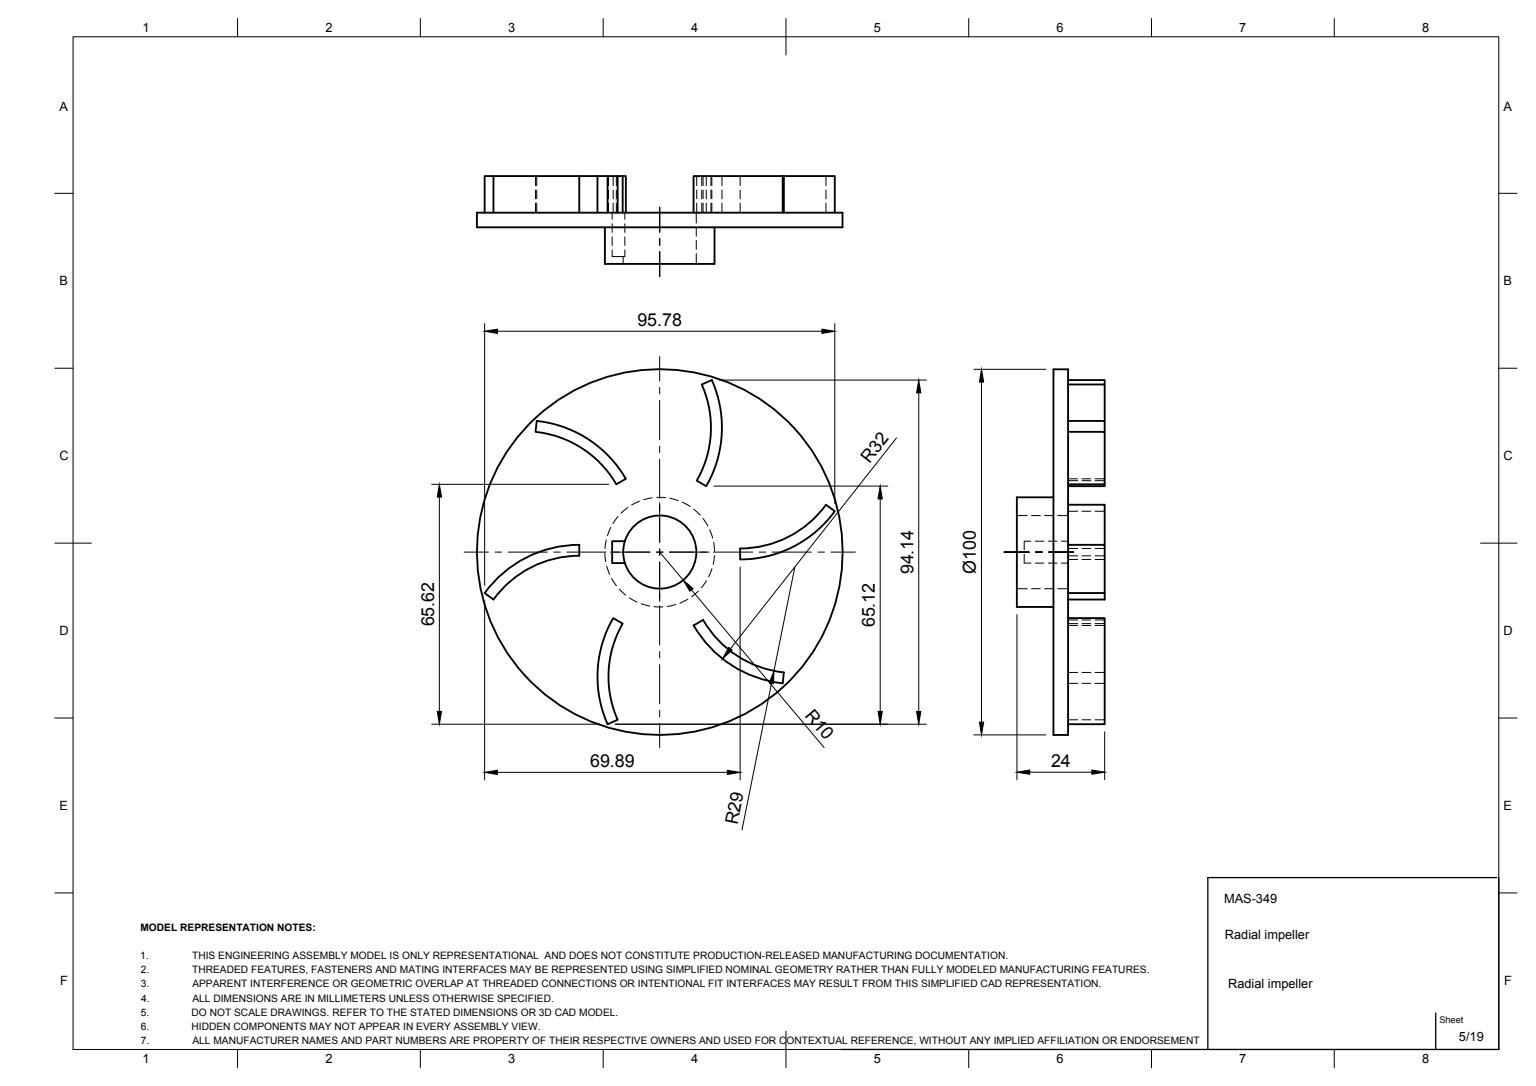
ISO-10303-21;
HEADER;
/* Generated by software containing ST-Developer
 * from STEP Tools, Inc. (www.steptools.com) 
 */

FILE_DESCRIPTION(
/* description */ ('Independent two-stage semi-open centrifugal-pump CAD. Shared impeller
s, open-machinable return casings, removable diaphragms, bronze wear/j
ournal rings, volume-preserving seal instances, retained keyed shaft, 
opposed mechanical face rings and partly threaded tie hardware. Native
 shaft rotation. Geometric topology/clearance only; flow/head/efficien
cy, pressure, cavitation, balance, preload, face loading and secondary
 seal fits/bonds, material/thermal/tolerance selection and life unassi
gned. External drive, coupling, anchors and piping bolts omitted.'),
/* implementation_level */ '2;1');

FILE_NAME(
/* name */ 'Radial impeller.step',
/* time_stamp */ '2026-11-08T18:06:32-08:00',
/* author */ (''),
/* organization */ (''),
/* preprocessor_version */ 'ST-DEVELOPER v20.2',
/* originating_system */ 'Autodesk Translation Framework v15.17.0.0',
/* authorisation */ '');

FILE_SCHEMA (('AUTOMOTIVE_DESIGN { 1 0 10303 214 3 1 1 }'));
ENDSEC;

DATA;
#10=MECHANICAL_DESIGN_GEOMETRIC_PRESENTATION_REPRESENTATION('',(#395),#16687);
#357=SHAPE_REPRESENTATION_RELATIONSHIP('SRR','None',#16766,#376);
#376=ADVANCED_BREP_SHAPE_REPRESENTATION('',(#414),#16670);
#395=STYLED_ITEM('',(#16870),#414);
#414=MANIFOLD_SOLID_BREP('Body1',#6114);
#466=FACE_BOUND('',#1139,.T.);
#467=FACE_BOUND('',#1140,.T.);
#468=FACE_BOUND('',#1141,.T.);
#469=FACE_BOUND('',#1142,.T.);
#470=FACE_BOUND('',#1143,.T.);
#471=FACE_BOUND('',#1144,.T.);
#472=FACE_BOUND('',#1145,.T.);
#473=FACE_BOUND('',#1178,.T.);
#474=FACE_BOUND('',#1182,.T.);
#587=PLANE('',#6481);
#588=PLANE('',#6482);
#589=PLANE('',#6483);
#590=PLANE('',#6484);
#591=PLANE('',#6486);
#592=PLANE('',#6504);
#593=PLANE('',#6507);
#594=PLANE('',#6508);
#595=PLANE('',#6511);
#596=PLANE('',#6514);
#597=PLANE('',#6515);
#598=PLANE('',#6518);
#599=PLANE('',#6521);
#600=PLANE('',#6522);
#601=PLANE('',#6525);
#602=PLANE('',#6528);
#603=PLANE('',#6529);
#604=PLANE('',#6532);
#605=PLANE('',#6535);
#606=PLANE('',#6536);
#607=PLANE('',#6539);
#608=PLANE('',#6542);
#609=PLANE('',#6543);
#610=PLANE('',#6547);
#611=PLANE('',#6552);
#752=FACE_OUTER_BOUND('',#1134,.T.);
#753=FACE_OUTER_BOUND('',#1135,.T.);
#754=FACE_OUTER_BOUND('',#1136,.T.);
#755=FACE_OUTER_BOUND('',#1137,.T.);
#756=FACE_OUTER_BOUND('',#1138,.T.);
#757=FACE_OUTER_BOUND('',#1146,.T.);
#758=FACE_OUTER_BOUND('',#1147,.T.);
#759=FACE_OUTER_BOUND('',#1148,.T.);
#760=FACE_OUTER_BOUND('',#1149,.T.);
#761=FACE_OUTER_BOUND('',#1150,.T.);
#762=FACE_OUTER_BOUND('',#1151,.T.);
#763=FACE_OUTER_BOUND('',#1152,.T.);
#764=FACE_OUTER_BOUND('',#1153,.T.);
#765=FACE_OUTER_BOUND('',#1154,.T.);
#766=FACE_OUTER_BOUND('',#1155,.T.);
#767=FACE_OUTER_BOUND('',#1156,.T.);
#768=FACE_OUTER_BOUND('',#1157,.T.);
#769=FACE_OUTER_BOUND('',#1158,.T.);
#770=FACE_OUTER_BOUND('',#1159,.T.);
#771=FACE_OUTER_BOUND('',#1160,.T.);
#772=FACE_OUTER_BOUND('',#1161,.T.);
#773=FACE_OUTER_BOUND('',#1162,.T.);
#774=FACE_OUTER_BOUND('',#1163,.T.);
#775=FACE_OUTER_BOUND('',#1164,.T.);
#776=FACE_OUTER_BOUND('',#1165,.T.);
#777=FACE_OUTER_BOUND('',#1166,.T.);
#778=FACE_OUTER_BOUND('',#1167,.T.);
#779=FACE_OUTER_BOUND('',#1168,.T.);
#780=FACE_OUTER_BOUND('',#1169,.T.);
#781=FACE_OUTER_BOUND('',#1170,.T.);
#782=FACE_OUTER_BOUND('',#1171,.T.);
#783=FACE_OUTER_BOUND('',#1172,.T.);
#784=FACE_OUTER_BOUND('',#1173,.T.);
#785=FACE_OUTER_BOUND('',#1174,.T.);
#786=FACE_OUTER_BOUND('',#1175,.T.);
#787=FACE_OUTER_BOUND('',#1176,.T.);
#788=FACE_OUTER_BOUND('',#1177,.T.);
#789=FACE_OUTER_BOUND('',#1179,.T.);
#790=FACE_OUTER_BOUND('',#1180,.T.);
#791=FACE_OUTER_BOUND('',#1181,.T.);
#1134=EDGE_LOOP('',(#4209,#4210,#4211,#4212));
#1135=EDGE_LOOP('',(#4213,#4214,#4215,#4216));
#1136=EDGE_LOOP('',(#4217,#4218,#4219,#4220));
#1137=EDGE_LOOP('',(#4221,#4222,#4223,#4224));
#1138=EDGE_LOOP('',(#4225));
#1139=EDGE_LOOP('',(#4226,#4227,#4228,#4229));
#1140=EDGE_LOOP('',(#4230,#4231,#4232,#4233));
#1141=EDGE_LOOP('',(#4234,#4235,#4236,#4237));
#1142=EDGE_LOOP('',(#4238,#4239,#4240,#4241));
#1143=EDGE_LOOP('',(#4242,#4243,#4244,#4245));
#1144=EDGE_LOOP('',(#4246,#4247,#4248,#4249));
#1145=EDGE_LOOP('',(#4250,#4251,#4252,#4253,#4254));
#1146=EDGE_LOOP('',(#4255,#4256,#4257,#4258));
#1147=EDGE_LOOP('',(#4259,#4260,#4261,#4262));
#1148=EDGE_LOOP('',(#4263,#4264,#4265,#4266));
#1149=EDGE_LOOP('',(#4267,#4268,#4269,#4270));
#1150=EDGE_LOOP('',(#4271,#4272,#4273,#4274));
#1151=EDGE_LOOP('',(#4275,#4276,#4277,#4278));
#1152=EDGE_LOOP('',(#4279,#4280,#4281,#4282));
#1153=EDGE_LOOP('',(#4283,#4284,#4285,#4286));
#1154=EDGE_LOOP('',(#4287,#4288,#4289,#4290));
#1155=EDGE_LOOP('',(#4291,#4292,#4293,#4294));
#1156=EDGE_LOOP('',(#4295,#4296,#4297,#4298));
#1157=EDGE_LOOP('',(#4299,#4300,#4301,#4302));
#1158=EDGE_LOOP('',(#4303,#4304,#4305,#4306));
#1159=EDGE_LOOP('',(#4307,#4308,#4309,#4310));
#1160=EDGE_LOOP('',(#4311,#4312,#4313,#4314));
#1161=EDGE_LOOP('',(#4315,#4316,#4317,#4318));
#1162=EDGE_LOOP('',(#4319,#4320,#4321,#4322));
#1163=EDGE_LOOP('',(#4323,#4324,#4325,#4326));
#1164=EDGE_LOOP('',(#4327,#4328,#4329,#4330));
#1165=EDGE_LOOP('',(#4331,#4332,#4333,#4334));
#1166=EDGE_LOOP('',(#4335,#4336,#4337,#4338));
#1167=EDGE_LOOP('',(#4339,#4340,#4341,#4342));
#1168=EDGE_LOOP('',(#4343,#4344,#4345,#4346));
#1169=EDGE_LOOP('',(#4347,#4348,#4349,#4350));
#1170=EDGE_LOOP('',(#4351,#4352,#4353,#4354));
#1171=EDGE_LOOP('',(#4355,#4356,#4357,#4358));
#1172=EDGE_LOOP('',(#4359,#4360,#4361,#4362));
#1173=EDGE_LOOP('',(#4363,#4364,#4365,#4366));
#1174=EDGE_LOOP('',(#4367,#4368,#4369,#4370));
#1175=EDGE_LOOP('',(#4371,#4372,#4373,#4374));
#1176=EDGE_LOOP('',(#4375,#4376,#4377,#4378));
#1177=EDGE_LOOP('',(#4379));
#1178=EDGE_LOOP('',(#4380));
#1179=EDGE_LOOP('',(#4381,#4382,#4383,#4384,#4385,#4386,#4387,#4388));
#1180=EDGE_LOOP('',(#4389,#4390,#4391,#4392));
#1181=EDGE_LOOP('',(#4393));
#1182=EDGE_LOOP('',(#4394));
#1591=LINE('',#8989,#1960);
#1592=LINE('',#8991,#1961);
#1593=LINE('',#8993,#1962);
#1594=LINE('',#8994,#1963);
#1595=LINE('',#8997,#1964);
#1596=LINE('',#8999,#1965);
#1597=LINE('',#9000,#1966);
#1598=LINE('',#9004,#1967);
#1599=LINE('',#9005,#1968);
#1600=LINE('',#9006,#1969);
#1601=LINE('',#9016,#1970);
#1602=LINE('',#9019,#1971);
#1603=LINE('',#9024,#1972);
#1604=LINE('',#9027,#1973);
#1605=LINE('',#9032,#1974);
#1606=LINE('',#9035,#1975);
#1607=LINE('',#9040,#1976);
#1608=LINE('',#9043,#1977);
#1609=LINE('',#9048,#1978);
#1610=LINE('',#9051,#1979);
#1611=LINE('',#9056,#1980);
#1612=LINE('',#9059,#1981);
#1613=LINE('',#9067,#1982);
#1614=LINE('',#9068,#1983);
#1615=LINE('',#9071,#1984);
#1616=LINE('',#9072,#1985);
#1617=LINE('',#9076,#1986);
#1618=LINE('',#9078,#1987);
#1619=LINE('',#9084,#1988);
#1620=LINE('',#9085,#1989);
#1621=LINE('',#9088,#1990);
#1622=LINE('',#9089,#1991);
#1623=LINE('',#9093,#1992);
#1624=LINE('',#9095,#1993);
#1625=LINE('',#9101,#1994);
#1626=LINE('',#9102,#1995);
#1627=LINE('',#9105,#1996);
#1628=LINE('',#9106,#1997);
#1629=LINE('',#9110,#1998);
#1630=LINE('',#9112,#1999);
#1631=LINE('',#9118,#2000);
#1632=LINE('',#9119,#2001);
#1633=LINE('',#9122,#2002);
#1634=LINE('',#9123,#2003);
#1635=LINE('',#9127,#2004);
#1636=LINE('',#9129,#2005);
#1637=LINE('',#9135,#2006);
#1638=LINE('',#9136,#2007);
#1639=LINE('',#9139,#2008);
#1640=LINE('',#9140,#2009);
#1641=LINE('',#9144,#2010);
#1642=LINE('',#9146,#2011);
#1643=LINE('',#9152,#2012);
#1644=LINE('',#9153,#2013);
#1645=LINE('',#9156,#2014);
#1646=LINE('',#9157,#2015);
#1647=LINE('',#9161,#2016);
#1648=LINE('',#9163,#2017);
#1649=LINE('',#9169,#2018);
#1650=LINE('',#9175,#2019);
#1651=LINE('',#9179,#2020);
#1960=VECTOR('',#7359,1.);
#1961=VECTOR('',#7360,1.);
#1962=VECTOR('',#7361,1.);
#1963=VECTOR('',#7362,1.);
#1964=VECTOR('',#7365,1.);
#1965=VECTOR('',#7366,1.);
#1966=VECTOR('',#7367,1.);
#1967=VECTOR('',#7370,1.);
#1968=VECTOR('',#7371,1.);
#1969=VECTOR('',#7372,1.);
#1970=VECTOR('',#7383,1.);
#1971=VECTOR('',#7386,1.);
#1972=VECTOR('',#7389,1.);
#1973=VECTOR('',#7392,1.);
#1974=VECTOR('',#7395,1.);
#1975=VECTOR('',#7398,1.);
#1976=VECTOR('',#7401,1.);
#1977=VECTOR('',#7404,1.);
#1978=VECTOR('',#7407,1.);
#1979=VECTOR('',#7410,1.);
#1980=VECTOR('',#7413,1.);
#1981=VECTOR('',#7416,1.);
#1982=VECTOR('',#7425,1.);
#1983=VECTOR('',#7426,1.);
#1984=VECTOR('',#7429,1.);
#1985=VECTOR('',#7430,1.);
#1986=VECTOR('',#7435,1.);
#1987=VECTOR('',#7438,1.);
#1988=VECTOR('',#7445,1.);
#1989=VECTOR('',#7446,1.);
#1990=VECTOR('',#7449,1.);
#1991=VECTOR('',#7450,1.);
#1992=VECTOR('',#7455,1.);
#1993=VECTOR('',#7458,1.);
#1994=VECTOR('',#7465,1.);
#1995=VECTOR('',#7466,1.);
#1996=VECTOR('',#7469,1.);
#1997=VECTOR('',#7470,1.);
#1998=VECTOR('',#7475,1.);
#1999=VECTOR('',#7478,1.);
#2000=VECTOR('',#7485,1.);
#2001=VECTOR('',#7486,1.);
#2002=VECTOR('',#7489,1.);
#2003=VECTOR('',#7490,1.);
#2004=VECTOR('',#7495,1.);
#2005=VECTOR('',#7498,1.);
#2006=VECTOR('',#7505,1.);
#2007=VECTOR('',#7506,1.);
#2008=VECTOR('',#7509,1.);
#2009=VECTOR('',#7510,1.);
#2010=VECTOR('',#7515,1.);
#2011=VECTOR('',#7518,1.);
#2012=VECTOR('',#7525,1.);
#2013=VECTOR('',#7526,1.);
#2014=VECTOR('',#7529,1.);
#2015=VECTOR('',#7530,1.);
#2016=VECTOR('',#7535,1.);
#2017=VECTOR('',#7538,1.);
#2018=VECTOR('',#7545,1.5);
#2019=VECTOR('',#7554,1.);
#2020=VECTOR('',#7559,5.);
#2310=CIRCLE('',#6485,1.);
#2311=CIRCLE('',#6487,5.);
#2312=CIRCLE('',#6488,2.9);
#2313=CIRCLE('',#6489,3.2);
#2314=CIRCLE('',#6490,2.9);
#2315=CIRCLE('',#6491,3.2);
#2316=CIRCLE('',#6492,2.9);
#2317=CIRCLE('',#6493,3.2);
#2318=CIRCLE('',#6494,2.9);
#2319=CIRCLE('',#6495,3.2);
#2320=CIRCLE('',#6496,2.9);
#2321=CIRCLE('',#6497,3.2);
#2322=CIRCLE('',#6498,2.9);
#2323=CIRCLE('',#6499,3.2);
#2324=CIRCLE('',#6500,1.);
#2325=CIRCLE('',#6501,1.);
#2326=CIRCLE('',#6503,2.9);
#2327=CIRCLE('',#6506,3.2);
#2328=CIRCLE('',#6510,2.9);
#2329=CIRCLE('',#6513,3.2);
#2330=CIRCLE('',#6517,2.9);
#2331=CIRCLE('',#6520,3.2);
#2332=CIRCLE('',#6524,2.9);
#2333=CIRCLE('',#6527,3.2);
#2334=CIRCLE('',#6531,2.9);
#2335=CIRCLE('',#6534,3.2);
#2336=CIRCLE('',#6538,2.9);
#2337=CIRCLE('',#6541,3.2);
#2338=CIRCLE('',#6545,1.5);
#2339=CIRCLE('',#6546,1.5);
#2340=CIRCLE('',#6548,1.);
#2341=CIRCLE('',#6551,5.);
#2605=VERTEX_POINT('',#8987);
#2606=VERTEX_POINT('',#8988);
#2607=VERTEX_POINT('',#8990);
#2608=VERTEX_POINT('',#8992);
#2609=VERTEX_POINT('',#8996);
#2610=VERTEX_POINT('',#8998);
#2611=VERTEX_POINT('',#9002);
#2612=VERTEX_POINT('',#9003);
#2613=VERTEX_POINT('',#9010);
#2614=VERTEX_POINT('',#9012);
#2615=VERTEX_POINT('',#9013);
#2616=VERTEX_POINT('',#9015);
#2617=VERTEX_POINT('',#9017);
#2618=VERTEX_POINT('',#9020);
#2619=VERTEX_POINT('',#9021);
#2620=VERTEX_POINT('',#9023);
#2621=VERTEX_POINT('',#9025);
#2622=VERTEX_POINT('',#9028);
#2623=VERTEX_POINT('',#9029);
#2624=VERTEX_POINT('',#9031);
#2625=VERTEX_POINT('',#9033);
#2626=VERTEX_POINT('',#9036);
#2627=VERTEX_POINT('',#9037);
#2628=VERTEX_POINT('',#9039);
#2629=VERTEX_POINT('',#9041);
#2630=VERTEX_POINT('',#9044);
#2631=VERTEX_POINT('',#9045);
#2632=VERTEX_POINT('',#9047);
#2633=VERTEX_POINT('',#9049);
#2634=VERTEX_POINT('',#9052);
#2635=VERTEX_POINT('',#9053);
#2636=VERTEX_POINT('',#9055);
#2637=VERTEX_POINT('',#9057);
#2638=VERTEX_POINT('',#9060);
#2639=VERTEX_POINT('',#9064);
#2640=VERTEX_POINT('',#9065);
#2641=VERTEX_POINT('',#9070);
#2642=VERTEX_POINT('',#9074);
#2643=VERTEX_POINT('',#9081);
#2644=VERTEX_POINT('',#9082);
#2645=VERTEX_POINT('',#9087);
#2646=VERTEX_POINT('',#9091);
#2647=VERTEX_POINT('',#9098);
#2648=VERTEX_POINT('',#9099);
#2649=VERTEX_POINT('',#9104);
#2650=VERTEX_POINT('',#9108);
#2651=VERTEX_POINT('',#9115);
#2652=VERTEX_POINT('',#9116);
#2653=VERTEX_POINT('',#9121);
#2654=VERTEX_POINT('',#9125);
#2655=VERTEX_POINT('',#9132);
#2656=VERTEX_POINT('',#9133);
#2657=VERTEX_POINT('',#9138);
#2658=VERTEX_POINT('',#9142);
#2659=VERTEX_POINT('',#9149);
#2660=VERTEX_POINT('',#9150);
#2661=VERTEX_POINT('',#9155);
#2662=VERTEX_POINT('',#9159);
#2663=VERTEX_POINT('',#9166);
#2664=VERTEX_POINT('',#9168);
#2665=VERTEX_POINT('',#9172);
#2666=VERTEX_POINT('',#9177);
#3214=EDGE_CURVE('',#2605,#2606,#1591,.T.);
#3215=EDGE_CURVE('',#2605,#2607,#1592,.T.);
#3216=EDGE_CURVE('',#2607,#2608,#1593,.T.);
#3217=EDGE_CURVE('',#2606,#2608,#1594,.T.);
#3218=EDGE_CURVE('',#2607,#2609,#1595,.T.);
#3219=EDGE_CURVE('',#2609,#2610,#1596,.T.);
#3220=EDGE_CURVE('',#2608,#2610,#1597,.T.);
#3221=EDGE_CURVE('',#2611,#2612,#1598,.T.);
#3222=EDGE_CURVE('',#2610,#2611,#1599,.T.);
#3223=EDGE_CURVE('',#2609,#2612,#1600,.T.);
#3224=EDGE_CURVE('',#2612,#2605,#2310,.T.);
#3225=EDGE_CURVE('',#2613,#2613,#2311,.T.);
#3226=EDGE_CURVE('',#2614,#2615,#2312,.T.);
#3227=EDGE_CURVE('',#2615,#2616,#1601,.T.);
#3228=EDGE_CURVE('',#2616,#2617,#2313,.T.);
#3229=EDGE_CURVE('',#2617,#2614,#1602,.T.);
#3230=EDGE_CURVE('',#2618,#2619,#2314,.T.);
#3231=EDGE_CURVE('',#2619,#2620,#1603,.T.);
#3232=EDGE_CURVE('',#2620,#2621,#2315,.T.);
#3233=EDGE_CURVE('',#2621,#2618,#1604,.T.);
#3234=EDGE_CURVE('',#2622,#2623,#2316,.T.);
#3235=EDGE_CURVE('',#2623,#2624,#1605,.T.);
#3236=EDGE_CURVE('',#2624,#2625,#2317,.T.);
#3237=EDGE_CURVE('',#2625,#2622,#1606,.T.);
#3238=EDGE_CURVE('',#2626,#2627,#2318,.T.);
#3239=EDGE_CURVE('',#2627,#2628,#1607,.T.);
#3240=EDGE_CURVE('',#2628,#2629,#2319,.T.);
#3241=EDGE_CURVE('',#2629,#2626,#1608,.T.);
#3242=EDGE_CURVE('',#2630,#2631,#2320,.T.);
#3243=EDGE_CURVE('',#2631,#2632,#1609,.T.);
#3244=EDGE_CURVE('',#2632,#2633,#2321,.T.);
#3245=EDGE_CURVE('',#2633,#2630,#1610,.T.);
#3246=EDGE_CURVE('',#2634,#2635,#2322,.T.);
#3247=EDGE_CURVE('',#2635,#2636,#1611,.T.);
#3248=EDGE_CURVE('',#2636,#2637,#2323,.T.);
#3249=EDGE_CURVE('',#2637,#2634,#1612,.T.);
#3250=EDGE_CURVE('',#2638,#2611,#2324,.T.);
#3251=EDGE_CURVE('',#2606,#2638,#2325,.T.);
#3252=EDGE_CURVE('',#2639,#2640,#2326,.T.);
#3253=EDGE_CURVE('',#2639,#2615,#1613,.T.);
#3254=EDGE_CURVE('',#2640,#2614,#1614,.T.);
#3255=EDGE_CURVE('',#2641,#2640,#1615,.T.);
#3256=EDGE_CURVE('',#2641,#2617,#1616,.T.);
#3257=EDGE_CURVE('',#2642,#2641,#2327,.T.);
#3258=EDGE_CURVE('',#2642,#2616,#1617,.T.);
#3259=EDGE_CURVE('',#2639,#2642,#1618,.T.);
#3260=EDGE_CURVE('',#2643,#2644,#2328,.T.);
#3261=EDGE_CURVE('',#2643,#2619,#1619,.T.);
#3262=EDGE_CURVE('',#2644,#2618,#1620,.T.);
#3263=EDGE_CURVE('',#2645,#2644,#1621,.T.);
#3264=EDGE_CURVE('',#2645,#2621,#1622,.T.);
#3265=EDGE_CURVE('',#2646,#2645,#2329,.T.);
#3266=EDGE_CURVE('',#2646,#2620,#1623,.T.);
#3267=EDGE_CURVE('',#2643,#2646,#1624,.T.);
#3268=EDGE_CURVE('',#2647,#2648,#2330,.T.);
#3269=EDGE_CURVE('',#2647,#2623,#1625,.T.);
#3270=EDGE_CURVE('',#2648,#2622,#1626,.T.);
#3271=EDGE_CURVE('',#2649,#2648,#1627,.T.);
#3272=EDGE_CURVE('',#2649,#2625,#1628,.T.);
#3273=EDGE_CURVE('',#2650,#2649,#2331,.T.);
#3274=EDGE_CURVE('',#2650,#2624,#1629,.T.);
#3275=EDGE_CURVE('',#2647,#2650,#1630,.T.);
#3276=EDGE_CURVE('',#2651,#2652,#2332,.T.);
#3277=EDGE_CURVE('',#2651,#2627,#1631,.T.);
#3278=EDGE_CURVE('',#2652,#2626,#1632,.T.);
#3279=EDGE_CURVE('',#2653,#2652,#1633,.T.);
#3280=EDGE_CURVE('',#2653,#2629,#1634,.T.);
#3281=EDGE_CURVE('',#2654,#2653,#2333,.T.);
#3282=EDGE_CURVE('',#2654,#2628,#1635,.T.);
#3283=EDGE_CURVE('',#2651,#2654,#1636,.T.);
#3284=EDGE_CURVE('',#2655,#2656,#2334,.T.);
#3285=EDGE_CURVE('',#2655,#2631,#1637,.T.);
#3286=EDGE_CURVE('',#2656,#2630,#1638,.T.);
#3287=EDGE_CURVE('',#2657,#2656,#1639,.T.);
#3288=EDGE_CURVE('',#2657,#2633,#1640,.T.);
#3289=EDGE_CURVE('',#2658,#2657,#2335,.T.);
#3290=EDGE_CURVE('',#2658,#2632,#1641,.T.);
#3291=EDGE_CURVE('',#2655,#2658,#1642,.T.);
#3292=EDGE_CURVE('',#2659,#2660,#2336,.T.);
#3293=EDGE_CURVE('',#2659,#2635,#1643,.T.);
#3294=EDGE_CURVE('',#2660,#2634,#1644,.T.);
#3295=EDGE_CURVE('',#2661,#2660,#1645,.T.);
#3296=EDGE_CURVE('',#2661,#2637,#1646,.T.);
#3297=EDGE_CURVE('',#2662,#2661,#2337,.T.);
#3298=EDGE_CURVE('',#2662,#2636,#1647,.T.);
#3299=EDGE_CURVE('',#2659,#2662,#1648,.T.);
#3300=EDGE_CURVE('',#2663,#2663,#2338,.T.);
#3301=EDGE_CURVE('',#2663,#2664,#1649,.T.);
#3302=EDGE_CURVE('',#2664,#2664,#2339,.T.);
#3303=EDGE_CURVE('',#2665,#2665,#2340,.T.);
#3304=EDGE_CURVE('',#2665,#2638,#1650,.T.);
#3305=EDGE_CURVE('',#2666,#2666,#2341,.T.);
#3306=EDGE_CURVE('',#2666,#2613,#1651,.T.);
#4209=ORIENTED_EDGE('',*,*,#3214,.F.);
#4210=ORIENTED_EDGE('',*,*,#3215,.T.);
#4211=ORIENTED_EDGE('',*,*,#3216,.T.);
#4212=ORIENTED_EDGE('',*,*,#3217,.F.);
#4213=ORIENTED_EDGE('',*,*,#3218,.T.);
#4214=ORIENTED_EDGE('',*,*,#3219,.T.);
#4215=ORIENTED_EDGE('',*,*,#3220,.F.);
#4216=ORIENTED_EDGE('',*,*,#3216,.F.);
#4217=ORIENTED_EDGE('',*,*,#3221,.F.);
#4218=ORIENTED_EDGE('',*,*,#3222,.F.);
#4219=ORIENTED_EDGE('',*,*,#3219,.F.);
#4220=ORIENTED_EDGE('',*,*,#3223,.T.);
#4221=ORIENTED_EDGE('',*,*,#3224,.F.);
#4222=ORIENTED_EDGE('',*,*,#3223,.F.);
#4223=ORIENTED_EDGE('',*,*,#3218,.F.);
#4224=ORIENTED_EDGE('',*,*,#3215,.F.);
#4225=ORIENTED_EDGE('',*,*,#3225,.F.);
#4226=ORIENTED_EDGE('',*,*,#3226,.T.);
#4227=ORIENTED_EDGE('',*,*,#3227,.T.);
#4228=ORIENTED_EDGE('',*,*,#3228,.T.);
#4229=ORIENTED_EDGE('',*,*,#3229,.T.);
#4230=ORIENTED_EDGE('',*,*,#3230,.T.);
#4231=ORIENTED_EDGE('',*,*,#3231,.T.);
#4232=ORIENTED_EDGE('',*,*,#3232,.T.);
#4233=ORIENTED_EDGE('',*,*,#3233,.T.);
#4234=ORIENTED_EDGE('',*,*,#3234,.T.);
#4235=ORIENTED_EDGE('',*,*,#3235,.T.);
#4236=ORIENTED_EDGE('',*,*,#3236,.T.);
#4237=ORIENTED_EDGE('',*,*,#3237,.T.);
#4238=ORIENTED_EDGE('',*,*,#3238,.T.);
#4239=ORIENTED_EDGE('',*,*,#3239,.T.);
#4240=ORIENTED_EDGE('',*,*,#3240,.T.);
#4241=ORIENTED_EDGE('',*,*,#3241,.T.);
#4242=ORIENTED_EDGE('',*,*,#3242,.T.);
#4243=ORIENTED_EDGE('',*,*,#3243,.T.);
#4244=ORIENTED_EDGE('',*,*,#3244,.T.);
#4245=ORIENTED_EDGE('',*,*,#3245,.T.);
#4246=ORIENTED_EDGE('',*,*,#3246,.T.);
#4247=ORIENTED_EDGE('',*,*,#3247,.T.);
#4248=ORIENTED_EDGE('',*,*,#3248,.T.);
#4249=ORIENTED_EDGE('',*,*,#3249,.T.);
#4250=ORIENTED_EDGE('',*,*,#3217,.T.);
#4251=ORIENTED_EDGE('',*,*,#3220,.T.);
#4252=ORIENTED_EDGE('',*,*,#3222,.T.);
#4253=ORIENTED_EDGE('',*,*,#3250,.F.);
#4254=ORIENTED_EDGE('',*,*,#3251,.F.);
#4255=ORIENTED_EDGE('',*,*,#3252,.F.);
#4256=ORIENTED_EDGE('',*,*,#3253,.T.);
#4257=ORIENTED_EDGE('',*,*,#3226,.F.);
#4258=ORIENTED_EDGE('',*,*,#3254,.F.);
#4259=ORIENTED_EDGE('',*,*,#3255,.T.);
#4260=ORIENTED_EDGE('',*,*,#3254,.T.);
#4261=ORIENTED_EDGE('',*,*,#3229,.F.);
#4262=ORIENTED_EDGE('',*,*,#3256,.F.);
#4263=ORIENTED_EDGE('',*,*,#3257,.T.);
#4264=ORIENTED_EDGE('',*,*,#3256,.T.);
#4265=ORIENTED_EDGE('',*,*,#3228,.F.);
#4266=ORIENTED_EDGE('',*,*,#3258,.F.);
#4267=ORIENTED_EDGE('',*,*,#3259,.T.);
#4268=ORIENTED_EDGE('',*,*,#3258,.T.);
#4269=ORIENTED_EDGE('',*,*,#3227,.F.);
#4270=ORIENTED_EDGE('',*,*,#3253,.F.);
#4271=ORIENTED_EDGE('',*,*,#3259,.F.);
#4272=ORIENTED_EDGE('',*,*,#3252,.T.);
#4273=ORIENTED_EDGE('',*,*,#3255,.F.);
#4274=ORIENTED_EDGE('',*,*,#3257,.F.);
#4275=ORIENTED_EDGE('',*,*,#3260,.F.);
#4276=ORIENTED_EDGE('',*,*,#3261,.T.);
#4277=ORIENTED_EDGE('',*,*,#3230,.F.);
#4278=ORIENTED_EDGE('',*,*,#3262,.F.);
#4279=ORIENTED_EDGE('',*,*,#3263,.T.);
#4280=ORIENTED_EDGE('',*,*,#3262,.T.);
#4281=ORIENTED_EDGE('',*,*,#3233,.F.);
#4282=ORIENTED_EDGE('',*,*,#3264,.F.);
#4283=ORIENTED_EDGE('',*,*,#3265,.T.);
#4284=ORIENTED_EDGE('',*,*,#3264,.T.);
#4285=ORIENTED_EDGE('',*,*,#3232,.F.);
#4286=ORIENTED_EDGE('',*,*,#3266,.F.);
#4287=ORIENTED_EDGE('',*,*,#3267,.T.);
#4288=ORIENTED_EDGE('',*,*,#3266,.T.);
#4289=ORIENTED_EDGE('',*,*,#3231,.F.);
#4290=ORIENTED_EDGE('',*,*,#3261,.F.);
#4291=ORIENTED_EDGE('',*,*,#3267,.F.);
#4292=ORIENTED_EDGE('',*,*,#3260,.T.);
#4293=ORIENTED_EDGE('',*,*,#3263,.F.);
#4294=ORIENTED_EDGE('',*,*,#3265,.F.);
#4295=ORIENTED_EDGE('',*,*,#3268,.F.);
#4296=ORIENTED_EDGE('',*,*,#3269,.T.);
#4297=ORIENTED_EDGE('',*,*,#3234,.F.);
#4298=ORIENTED_EDGE('',*,*,#3270,.F.);
#4299=ORIENTED_EDGE('',*,*,#3271,.T.);
#4300=ORIENTED_EDGE('',*,*,#3270,.T.);
#4301=ORIENTED_EDGE('',*,*,#3237,.F.);
#4302=ORIENTED_EDGE('',*,*,#3272,.F.);
#4303=ORIENTED_EDGE('',*,*,#3273,.T.);
#4304=ORIENTED_EDGE('',*,*,#3272,.T.);
#4305=ORIENTED_EDGE('',*,*,#3236,.F.);
#4306=ORIENTED_EDGE('',*,*,#3274,.F.);
#4307=ORIENTED_EDGE('',*,*,#3275,.T.);
#4308=ORIENTED_EDGE('',*,*,#3274,.T.);
#4309=ORIENTED_EDGE('',*,*,#3235,.F.);
#4310=ORIENTED_EDGE('',*,*,#3269,.F.);
#4311=ORIENTED_EDGE('',*,*,#3275,.F.);
#4312=ORIENTED_EDGE('',*,*,#3268,.T.);
#4313=ORIENTED_EDGE('',*,*,#3271,.F.);
#4314=ORIENTED_EDGE('',*,*,#3273,.F.);
#4315=ORIENTED_EDGE('',*,*,#3276,.F.);
#4316=ORIENTED_EDGE('',*,*,#3277,.T.);
#4317=ORIENTED_EDGE('',*,*,#3238,.F.);
#4318=ORIENTED_EDGE('',*,*,#3278,.F.);
#4319=ORIENTED_EDGE('',*,*,#3279,.T.);
#4320=ORIENTED_EDGE('',*,*,#3278,.T.);
#4321=ORIENTED_EDGE('',*,*,#3241,.F.);
#4322=ORIENTED_EDGE('',*,*,#3280,.F.);
#4323=ORIENTED_EDGE('',*,*,#3281,.T.);
#4324=ORIENTED_EDGE('',*,*,#3280,.T.);
#4325=ORIENTED_EDGE('',*,*,#3240,.F.);
#4326=ORIENTED_EDGE('',*,*,#3282,.F.);
#4327=ORIENTED_EDGE('',*,*,#3283,.T.);
#4328=ORIENTED_EDGE('',*,*,#3282,.T.);
#4329=ORIENTED_EDGE('',*,*,#3239,.F.);
#4330=ORIENTED_EDGE('',*,*,#3277,.F.);
#4331=ORIENTED_EDGE('',*,*,#3283,.F.);
#4332=ORIENTED_EDGE('',*,*,#3276,.T.);
#4333=ORIENTED_EDGE('',*,*,#3279,.F.);
#4334=ORIENTED_EDGE('',*,*,#3281,.F.);
#4335=ORIENTED_EDGE('',*,*,#3284,.F.);
#4336=ORIENTED_EDGE('',*,*,#3285,.T.);
#4337=ORIENTED_EDGE('',*,*,#3242,.F.);
#4338=ORIENTED_EDGE('',*,*,#3286,.F.);
#4339=ORIENTED_EDGE('',*,*,#3287,.T.);
#4340=ORIENTED_EDGE('',*,*,#3286,.T.);
#4341=ORIENTED_EDGE('',*,*,#3245,.F.);
#4342=ORIENTED_EDGE('',*,*,#3288,.F.);
#4343=ORIENTED_EDGE('',*,*,#3289,.T.);
#4344=ORIENTED_EDGE('',*,*,#3288,.T.);
#4345=ORIENTED_EDGE('',*,*,#3244,.F.);
#4346=ORIENTED_EDGE('',*,*,#3290,.F.);
#4347=ORIENTED_EDGE('',*,*,#3291,.T.);
#4348=ORIENTED_EDGE('',*,*,#3290,.T.);
#4349=ORIENTED_EDGE('',*,*,#3243,.F.);
#4350=ORIENTED_EDGE('',*,*,#3285,.F.);
#4351=ORIENTED_EDGE('',*,*,#3291,.F.);
#4352=ORIENTED_EDGE('',*,*,#3284,.T.);
#4353=ORIENTED_EDGE('',*,*,#3287,.F.);
#4354=ORIENTED_EDGE('',*,*,#3289,.F.);
#4355=ORIENTED_EDGE('',*,*,#3292,.F.);
#4356=ORIENTED_EDGE('',*,*,#3293,.T.);
#4357=ORIENTED_EDGE('',*,*,#3246,.F.);
#4358=ORIENTED_EDGE('',*,*,#3294,.F.);
#4359=ORIENTED_EDGE('',*,*,#3295,.T.);
#4360=ORIENTED_EDGE('',*,*,#3294,.T.);
#4361=ORIENTED_EDGE('',*,*,#3249,.F.);
#4362=ORIENTED_EDGE('',*,*,#3296,.F.);
#4363=ORIENTED_EDGE('',*,*,#3297,.T.);
#4364=ORIENTED_EDGE('',*,*,#3296,.T.);
#4365=ORIENTED_EDGE('',*,*,#3248,.F.);
#4366=ORIENTED_EDGE('',*,*,#3298,.F.);
#4367=ORIENTED_EDGE('',*,*,#3299,.T.);
#4368=ORIENTED_EDGE('',*,*,#3298,.T.);
#4369=ORIENTED_EDGE('',*,*,#3247,.F.);
#4370=ORIENTED_EDGE('',*,*,#3293,.F.);
#4371=ORIENTED_EDGE('',*,*,#3299,.F.);
#4372=ORIENTED_EDGE('',*,*,#3292,.T.);
#4373=ORIENTED_EDGE('',*,*,#3295,.F.);
#4374=ORIENTED_EDGE('',*,*,#3297,.F.);
#4375=ORIENTED_EDGE('',*,*,#3300,.F.);
#4376=ORIENTED_EDGE('',*,*,#3301,.T.);
#4377=ORIENTED_EDGE('',*,*,#3302,.F.);
#4378=ORIENTED_EDGE('',*,*,#3301,.F.);
#4379=ORIENTED_EDGE('',*,*,#3300,.T.);
#4380=ORIENTED_EDGE('',*,*,#3303,.T.);
#4381=ORIENTED_EDGE('',*,*,#3303,.F.);
#4382=ORIENTED_EDGE('',*,*,#3304,.T.);
#4383=ORIENTED_EDGE('',*,*,#3250,.T.);
#4384=ORIENTED_EDGE('',*,*,#3221,.T.);
#4385=ORIENTED_EDGE('',*,*,#3224,.T.);
#4386=ORIENTED_EDGE('',*,*,#3214,.T.);
#4387=ORIENTED_EDGE('',*,*,#3251,.T.);
#4388=ORIENTED_EDGE('',*,*,#3304,.F.);
#4389=ORIENTED_EDGE('',*,*,#3305,.F.);
#4390=ORIENTED_EDGE('',*,*,#3306,.T.);
#4391=ORIENTED_EDGE('',*,*,#3225,.T.);
#4392=ORIENTED_EDGE('',*,*,#3306,.F.);
#4393=ORIENTED_EDGE('',*,*,#3305,.T.);
#4394=ORIENTED_EDGE('',*,*,#3302,.T.);
#5595=CYLINDRICAL_SURFACE('',#6502,2.9);
#5596=CYLINDRICAL_SURFACE('',#6505,3.2);
#5597=CYLINDRICAL_SURFACE('',#6509,2.9);
#5598=CYLINDRICAL_SURFACE('',#6512,3.2);
#5599=CYLINDRICAL_SURFACE('',#6516,2.9);
#5600=CYLINDRICAL_SURFACE('',#6519,3.2);
#5601=CYLINDRICAL_SURFACE('',#6523,2.9);
#5602=CYLINDRICAL_SURFACE('',#6526,3.2);
#5603=CYLINDRICAL_SURFACE('',#6530,2.9);
#5604=CYLINDRICAL_SURFACE('',#6533,3.2);
#5605=CYLINDRICAL_SURFACE('',#6537,2.9);
#5606=CYLINDRICAL_SURFACE('',#6540,3.2);
#5607=CYLINDRICAL_SURFACE('',#6544,1.5);
#5608=CYLINDRICAL_SURFACE('',#6549,1.);
#5609=CYLINDRICAL_SURFACE('',#6550,5.);
#5831=ADVANCED_FACE('',(#752),#587,.F.);
#5832=ADVANCED_FACE('',(#753),#588,.F.);
#5833=ADVANCED_FACE('',(#754),#589,.F.);
#5834=ADVANCED_FACE('',(#755),#590,.F.);
#5835=ADVANCED_FACE('',(#756,#466,#467,#468,#469,#470,#471,#472),#591,.F.);
#5836=ADVANCED_FACE('',(#757),#5595,.F.);
#5837=ADVANCED_FACE('',(#758),#592,.T.);
#5838=ADVANCED_FACE('',(#759),#5596,.T.);
#5839=ADVANCED_FACE('',(#760),#593,.T.);
#5840=ADVANCED_FACE('',(#761),#594,.F.);
#5841=ADVANCED_FACE('',(#762),#5597,.F.);
#5842=ADVANCED_FACE('',(#763),#595,.T.);
#5843=ADVANCED_FACE('',(#764),#5598,.T.);
#5844=ADVANCED_FACE('',(#765),#596,.T.);
#5845=ADVANCED_FACE('',(#766),#597,.F.);
#5846=ADVANCED_FACE('',(#767),#5599,.F.);
#5847=ADVANCED_FACE('',(#768),#598,.T.);
#5848=ADVANCED_FACE('',(#769),#5600,.T.);
#5849=ADVANCED_FACE('',(#770),#599,.T.);
#5850=ADVANCED_FACE('',(#771),#600,.F.);
#5851=ADVANCED_FACE('',(#772),#5601,.F.);
#5852=ADVANCED_FACE('',(#773),#601,.T.);
#5853=ADVANCED_FACE('',(#774),#5602,.T.);
#5854=ADVANCED_FACE('',(#775),#602,.T.);
#5855=ADVANCED_FACE('',(#776),#603,.F.);
#5856=ADVANCED_FACE('',(#777),#5603,.F.);
#5857=ADVANCED_FACE('',(#778),#604,.T.);
#5858=ADVANCED_FACE('',(#779),#5604,.T.);
#5859=ADVANCED_FACE('',(#780),#605,.T.);
#5860=ADVANCED_FACE('',(#781),#606,.F.);
#5861=ADVANCED_FACE('',(#782),#5605,.F.);
#5862=ADVANCED_FACE('',(#783),#607,.T.);
#5863=ADVANCED_FACE('',(#784),#5606,.T.);
#5864=ADVANCED_FACE('',(#785),#608,.T.);
#5865=ADVANCED_FACE('',(#786),#609,.F.);
#5866=ADVANCED_FACE('',(#787),#5607,.T.);
#5867=ADVANCED_FACE('',(#788,#473),#610,.T.);
#5868=ADVANCED_FACE('',(#789),#5608,.F.);
#5869=ADVANCED_FACE('',(#790),#5609,.T.);
#5870=ADVANCED_FACE('',(#791,#474),#611,.T.);
#6114=CLOSED_SHELL('',(#5831,#5832,#5833,#5834,#5835,#5836,#5837,#5838,
#5839,#5840,#5841,#5842,#5843,#5844,#5845,#5846,#5847,#5848,#5849,#5850,
#5851,#5852,#5853,#5854,#5855,#5856,#5857,#5858,#5859,#5860,#5861,#5862,
#5863,#5864,#5865,#5866,#5867,#5868,#5869,#5870));
#6480=AXIS2_PLACEMENT_3D('',#8985,#7355,#7356);
#6481=AXIS2_PLACEMENT_3D('',#8986,#7357,#7358);
#6482=AXIS2_PLACEMENT_3D('',#8995,#7363,#7364);
#6483=AXIS2_PLACEMENT_3D('',#9001,#7368,#7369);
#6484=AXIS2_PLACEMENT_3D('',#9007,#7373,#7374);
#6485=AXIS2_PLACEMENT_3D('',#9008,#7375,#7376);
#6486=AXIS2_PLACEMENT_3D('',#9009,#7377,#7378);
#6487=AXIS2_PLACEMENT_3D('',#9011,#7379,#7380);
#6488=AXIS2_PLACEMENT_3D('',#9014,#7381,#7382);
#6489=AXIS2_PLACEMENT_3D('',#9018,#7384,#7385);
#6490=AXIS2_PLACEMENT_3D('',#9022,#7387,#7388);
#6491=AXIS2_PLACEMENT_3D('',#9026,#7390,#7391);
#6492=AXIS2_PLACEMENT_3D('',#9030,#7393,#7394);
#6493=AXIS2_PLACEMENT_3D('',#9034,#7396,#7397);
#6494=AXIS2_PLACEMENT_3D('',#9038,#7399,#7400);
#6495=AXIS2_PLACEMENT_3D('',#9042,#7402,#7403);
#6496=AXIS2_PLACEMENT_3D('',#9046,#7405,#7406);
#6497=AXIS2_PLACEMENT_3D('',#9050,#7408,#7409);
#6498=AXIS2_PLACEMENT_3D('',#9054,#7411,#7412);
#6499=AXIS2_PLACEMENT_3D('',#9058,#7414,#7415);
#6500=AXIS2_PLACEMENT_3D('',#9061,#7417,#7418);
#6501=AXIS2_PLACEMENT_3D('',#9062,#7419,#7420);
#6502=AXIS2_PLACEMENT_3D('',#9063,#7421,#7422);
#6503=AXIS2_PLACEMENT_3D('',#9066,#7423,#7424);
#6504=AXIS2_PLACEMENT_3D('',#9069,#7427,#7428);
#6505=AXIS2_PLACEMENT_3D('',#9073,#7431,#7432);
#6506=AXIS2_PLACEMENT_3D('',#9075,#7433,#7434);
#6507=AXIS2_PLACEMENT_3D('',#9077,#7436,#7437);
#6508=AXIS2_PLACEMENT_3D('',#9079,#7439,#7440);
#6509=AXIS2_PLACEMENT_3D('',#9080,#7441,#7442);
#6510=AXIS2_PLACEMENT_3D('',#9083,#7443,#7444);
#6511=AXIS2_PLACEMENT_3D('',#9086,#7447,#7448);
#6512=AXIS2_PLACEMENT_3D('',#9090,#7451,#7452);
#6513=AXIS2_PLACEMENT_3D('',#9092,#7453,#7454);
#6514=AXIS2_PLACEMENT_3D('',#9094,#7456,#7457);
#6515=AXIS2_PLACEMENT_3D('',#9096,#7459,#7460);
#6516=AXIS2_PLACEMENT_3D('',#9097,#7461,#7462);
#6517=AXIS2_PLACEMENT_3D('',#9100,#7463,#7464);
#6518=AXIS2_PLACEMENT_3D('',#9103,#7467,#7468);
#6519=AXIS2_PLACEMENT_3D('',#9107,#7471,#7472);
#6520=AXIS2_PLACEMENT_3D('',#9109,#7473,#7474);
#6521=AXIS2_PLACEMENT_3D('',#9111,#7476,#7477);
#6522=AXIS2_PLACEMENT_3D('',#9113,#7479,#7480);
#6523=AXIS2_PLACEMENT_3D('',#9114,#7481,#7482);
#6524=AXIS2_PLACEMENT_3D('',#9117,#7483,#7484);
#6525=AXIS2_PLACEMENT_3D('',#9120,#7487,#7488);
#6526=AXIS2_PLACEMENT_3D('',#9124,#7491,#7492);
#6527=AXIS2_PLACEMENT_3D('',#9126,#7493,#7494);
#6528=AXIS2_PLACEMENT_3D('',#9128,#7496,#7497);
#6529=AXIS2_PLACEMENT_3D('',#9130,#7499,#7500);
#6530=AXIS2_PLACEMENT_3D('',#9131,#7501,#7502);
#6531=AXIS2_PLACEMENT_3D('',#9134,#7503,#7504);
#6532=AXIS2_PLACEMENT_3D('',#9137,#7507,#7508);
#6533=AXIS2_PLACEMENT_3D('',#9141,#7511,#7512);
#6534=AXIS2_PLACEMENT_3D('',#9143,#7513,#7514);
#6535=AXIS2_PLACEMENT_3D('',#9145,#7516,#7517);
#6536=AXIS2_PLACEMENT_3D('',#9147,#7519,#7520);
#6537=AXIS2_PLACEMENT_3D('',#9148,#7521,#7522);
#6538=AXIS2_PLACEMENT_3D('',#9151,#7523,#7524);
#6539=AXIS2_PLACEMENT_3D('',#9154,#7527,#7528);
#6540=AXIS2_PLACEMENT_3D('',#9158,#7531,#7532);
#6541=AXIS2_PLACEMENT_3D('',#9160,#7533,#7534);
#6542=AXIS2_PLACEMENT_3D('',#9162,#7536,#7537);
#6543=AXIS2_PLACEMENT_3D('',#9164,#7539,#7540);
#6544=AXIS2_PLACEMENT_3D('',#9165,#7541,#7542);
#6545=AXIS2_PLACEMENT_3D('',#9167,#7543,#7544);
#6546=AXIS2_PLACEMENT_3D('',#9170,#7546,#7547);
#6547=AXIS2_PLACEMENT_3D('',#9171,#7548,#7549);
#6548=AXIS2_PLACEMENT_3D('',#9173,#7550,#7551);
#6549=AXIS2_PLACEMENT_3D('',#9174,#7552,#7553);
#6550=AXIS2_PLACEMENT_3D('',#9176,#7555,#7556);
#6551=AXIS2_PLACEMENT_3D('',#9178,#7557,#7558);
#6552=AXIS2_PLACEMENT_3D('',#9180,#7560,#7561);
#7355=DIRECTION('axis',(0.,0.,1.));
#7356=DIRECTION('refdir',(1.,0.,0.));
#7357=DIRECTION('center_axis',(0.,-1.,0.));
#7358=DIRECTION('ref_axis',(-1.,0.,0.));
#7359=DIRECTION('',(0.,0.,-1.));
#7360=DIRECTION('',(1.,0.,0.));
#7361=DIRECTION('',(0.,0.,-1.));
#7362=DIRECTION('',(1.,0.,0.));
#7363=DIRECTION('center_axis',(1.,0.,0.));
#7364=DIRECTION('ref_axis',(0.,-1.,0.));
#7365=DIRECTION('',(0.,1.,0.));
#7366=DIRECTION('',(0.,0.,-1.));
#7367=DIRECTION('',(0.,1.,0.));
#7368=DIRECTION('center_axis',(0.,1.,0.));
#7369=DIRECTION('ref_axis',(1.,0.,0.));
#7370=DIRECTION('',(0.,0.,1.));
#7371=DIRECTION('',(-1.,0.,0.));
#7372=DIRECTION('',(-1.,0.,0.));
#7373=DIRECTION('center_axis',(0.,0.,1.));
#7374=DIRECTION('ref_axis',(1.,0.,0.));
#7375=DIRECTION('center_axis',(0.,0.,-1.));
#7376=DIRECTION('ref_axis',(1.,0.,0.));
#7377=DIRECTION('center_axis',(0.,0.,1.));
#7378=DIRECTION('ref_axis',(1.,0.,0.));
#7379=DIRECTION('center_axis',(0.,0.,1.));
#7380=DIRECTION('ref_axis',(1.,0.,0.));
#7381=DIRECTION('center_axis',(0.,0.,-1.));
#7382=DIRECTION('ref_axis',(0.913545457642601,-0.406736643075801,0.));
#7383=DIRECTION('',(0.913545457642601,-0.406736643075801,0.));
#7384=DIRECTION('center_axis',(0.,0.,1.));
#7385=DIRECTION('ref_axis',(0.9135454576426,-0.406736643075801,0.));
#7386=DIRECTION('',(-0.866025403784439,-0.499999999999999,0.));
#7387=DIRECTION('center_axis',(0.,0.,-1.));
#7388=DIRECTION('ref_axis',(0.104528463267653,-0.994521895368273,0.));
#7389=DIRECTION('',(0.104528463267653,-0.994521895368273,0.));
#7390=DIRECTION('center_axis',(0.,0.,1.));
#7391=DIRECTION('ref_axis',(0.104528463267653,-0.994521895368274,0.));
#7392=DIRECTION('',(-0.866025403784438,0.5,0.));
#7393=DIRECTION('center_axis',(0.,0.,-1.));
#7394=DIRECTION('ref_axis',(-0.809016994374948,-0.587785252292473,0.));
#7395=DIRECTION('',(-0.809016994374947,-0.587785252292473,0.));
#7396=DIRECTION('center_axis',(0.,0.,1.));
#7397=DIRECTION('ref_axis',(-0.809016994374948,-0.587785252292473,0.));
#7398=DIRECTION('',(1.66533453693773E-16,1.,0.));
#7399=DIRECTION('center_axis',(0.,0.,-1.));
#7400=DIRECTION('ref_axis',(-0.913545457642601,0.406736643075801,0.));
#7401=DIRECTION('',(-0.913545457642601,0.4067366430758,0.));
#7402=DIRECTION('center_axis',(0.,0.,1.));
#7403=DIRECTION('ref_axis',(-0.913545457642601,0.406736643075801,0.));
#7404=DIRECTION('',(0.866025403784439,0.5,0.));
#7405=DIRECTION('center_axis',(0.,0.,-1.));
#7406=DIRECTION('ref_axis',(-0.104528463267653,0.994521895368273,0.));
#7407=DIRECTION('',(-0.104528463267653,0.994521895368273,0.));
#7408=DIRECTION('center_axis',(0.,0.,1.));
#7409=DIRECTION('ref_axis',(-0.104528463267653,0.994521895368273,0.));
#7410=DIRECTION('',(0.866025403784439,-0.5,0.));
#7411=DIRECTION('center_axis',(0.,0.,-1.));
#7412=DIRECTION('ref_axis',(0.809016994374948,0.587785252292473,0.));
#7413=DIRECTION('',(0.809016994374947,0.587785252292473,0.));
#7414=DIRECTION('center_axis',(0.,0.,1.));
#7415=DIRECTION('ref_axis',(0.809016994374948,0.587785252292473,0.));
#7416=DIRECTION('',(0.,-1.,0.));
#7417=DIRECTION('center_axis',(0.,0.,-1.));
#7418=DIRECTION('ref_axis',(1.,0.,0.));
#7419=DIRECTION('center_axis',(0.,0.,-1.));
#7420=DIRECTION('ref_axis',(1.,0.,0.));
#7421=DIRECTION('center_axis',(0.,0.,1.));
#7422=DIRECTION('ref_axis',(0.913545457642601,-0.406736643075801,0.));
#7423=DIRECTION('center_axis',(0.,0.,1.));
#7424=DIRECTION('ref_axis',(0.913545457642601,-0.406736643075801,0.));
#7425=DIRECTION('',(0.,0.,1.));
#7426=DIRECTION('',(0.,0.,1.));
#7427=DIRECTION('center_axis',(-0.499999999999999,0.866025403784439,0.));
#7428=DIRECTION('ref_axis',(-0.866025403784439,-0.499999999999999,0.));
#7429=DIRECTION('',(-0.866025403784439,-0.499999999999999,0.));
#7430=DIRECTION('',(0.,0.,1.));
#7431=DIRECTION('center_axis',(0.,0.,1.));
#7432=DIRECTION('ref_axis',(0.9135454576426,-0.406736643075801,0.));
#7433=DIRECTION('center_axis',(0.,0.,1.));
#7434=DIRECTION('ref_axis',(0.9135454576426,-0.406736643075801,0.));
#7435=DIRECTION('',(0.,0.,1.));
#7436=DIRECTION('center_axis',(-0.406736643075801,-0.913545457642601,0.));
#7437=DIRECTION('ref_axis',(0.913545457642601,-0.406736643075801,0.));
#7438=DIRECTION('',(0.913545457642601,-0.406736643075801,0.));
#7439=DIRECTION('center_axis',(0.,0.,1.));
#7440=DIRECTION('ref_axis',(0.499999999999999,-0.866025403784439,0.));
#7441=DIRECTION('center_axis',(0.,0.,1.));
#7442=DIRECTION('ref_axis',(0.104528463267653,-0.994521895368273,0.));
#7443=DIRECTION('center_axis',(0.,0.,1.));
#7444=DIRECTION('ref_axis',(0.104528463267653,-0.994521895368273,0.));
#7445=DIRECTION('',(0.,0.,1.));
#7446=DIRECTION('',(0.,0.,1.));
#7447=DIRECTION('center_axis',(0.5,0.866025403784438,0.));
#7448=DIRECTION('ref_axis',(-0.866025403784438,0.5,0.));
#7449=DIRECTION('',(-0.866025403784438,0.5,0.));
#7450=DIRECTION('',(0.,0.,1.));
#7451=DIRECTION('center_axis',(0.,0.,1.));
#7452=DIRECTION('ref_axis',(0.104528463267653,-0.994521895368274,0.));
#7453=DIRECTION('center_axis',(0.,0.,1.));
#7454=DIRECTION('ref_axis',(0.104528463267653,-0.994521895368274,0.));
#7455=DIRECTION('',(0.,0.,1.));
#7456=DIRECTION('center_axis',(-0.994521895368273,-0.104528463267653,0.));
#7457=DIRECTION('ref_axis',(0.104528463267653,-0.994521895368273,0.));
#7458=DIRECTION('',(0.104528463267653,-0.994521895368273,0.));
#7459=DIRECTION('center_axis',(0.,0.,1.));
#7460=DIRECTION('ref_axis',(-0.5,-0.866025403784438,0.));
#7461=DIRECTION('center_axis',(0.,0.,1.));
#7462=DIRECTION('ref_axis',(-0.809016994374948,-0.587785252292473,0.));
#7463=DIRECTION('center_axis',(0.,0.,1.));
#7464=DIRECTION('ref_axis',(-0.809016994374948,-0.587785252292473,0.));
#7465=DIRECTION('',(0.,0.,1.));
#7466=DIRECTION('',(0.,0.,1.));
#7467=DIRECTION('center_axis',(1.,-1.66533453693773E-16,0.));
#7468=DIRECTION('ref_axis',(1.66533453693773E-16,1.,0.));
#7469=DIRECTION('',(1.66533453693773E-16,1.,0.));
#7470=DIRECTION('',(0.,0.,1.));
#7471=DIRECTION('center_axis',(0.,0.,1.));
#7472=DIRECTION('ref_axis',(-0.809016994374948,-0.587785252292473,0.));
#7473=DIRECTION('center_axis',(0.,0.,1.));
#7474=DIRECTION('ref_axis',(-0.809016994374948,-0.587785252292473,0.));
#7475=DIRECTION('',(0.,0.,1.));
#7476=DIRECTION('center_axis',(-0.587785252292473,0.809016994374947,0.));
#7477=DIRECTION('ref_axis',(-0.809016994374947,-0.587785252292473,0.));
#7478=DIRECTION('',(-0.809016994374947,-0.587785252292473,0.));
#7479=DIRECTION('center_axis',(0.,0.,1.));
#7480=DIRECTION('ref_axis',(-1.,1.66533453693773E-16,0.));
#7481=DIRECTION('center_axis',(0.,0.,1.));
#7482=DIRECTION('ref_axis',(-0.913545457642601,0.406736643075801,0.));
#7483=DIRECTION('center_axis',(0.,0.,1.));
#7484=DIRECTION('ref_axis',(-0.913545457642601,0.406736643075801,0.));
#7485=DIRECTION('',(0.,0.,1.));
#7486=DIRECTION('',(0.,0.,1.));
#7487=DIRECTION('center_axis',(0.5,-0.866025403784439,0.));
#7488=DIRECTION('ref_axis',(0.866025403784439,0.5,0.));
#7489=DIRECTION('',(0.866025403784439,0.5,0.));
#7490=DIRECTION('',(0.,0.,1.));
#7491=DIRECTION('center_axis',(0.,0.,1.));
#7492=DIRECTION('ref_axis',(-0.913545457642601,0.406736643075801,0.));
#7493=DIRECTION('center_axis',(0.,0.,1.));
#7494=DIRECTION('ref_axis',(-0.913545457642601,0.406736643075801,0.));
#7495=DIRECTION('',(0.,0.,1.));
#7496=DIRECTION('center_axis',(0.4067366430758,0.913545457642601,0.));
#7497=DIRECTION('ref_axis',(-0.913545457642601,0.4067366430758,0.));
#7498=DIRECTION('',(-0.913545457642601,0.4067366430758,0.));
#7499=DIRECTION('center_axis',(0.,0.,1.));
#7500=DIRECTION('ref_axis',(-0.5,0.866025403784439,0.));
#7501=DIRECTION('center_axis',(0.,0.,1.));
#7502=DIRECTION('ref_axis',(-0.104528463267653,0.994521895368273,0.));
#7503=DIRECTION('center_axis',(0.,0.,1.));
#7504=DIRECTION('ref_axis',(-0.104528463267653,0.994521895368273,0.));
#7505=DIRECTION('',(0.,0.,1.));
#7506=DIRECTION('',(0.,0.,1.));
#7507=DIRECTION('center_axis',(-0.5,-0.866025403784439,0.));
#7508=DIRECTION('ref_axis',(0.866025403784439,-0.5,0.));
#7509=DIRECTION('',(0.866025403784439,-0.5,0.));
#7510=DIRECTION('',(0.,0.,1.));
#7511=DIRECTION('center_axis',(0.,0.,1.));
#7512=DIRECTION('ref_axis',(-0.104528463267653,0.994521895368273,0.));
#7513=DIRECTION('center_axis',(0.,0.,1.));
#7514=DIRECTION('ref_axis',(-0.104528463267653,0.994521895368273,0.));
#7515=DIRECTION('',(0.,0.,1.));
#7516=DIRECTION('center_axis',(0.994521895368273,0.104528463267653,0.));
#7517=DIRECTION('ref_axis',(-0.104528463267653,0.994521895368273,0.));
#7518=DIRECTION('',(-0.104528463267653,0.994521895368273,0.));
#7519=DIRECTION('center_axis',(0.,0.,1.));
#7520=DIRECTION('ref_axis',(0.5,0.866025403784439,0.));
#7521=DIRECTION('center_axis',(0.,0.,1.));
#7522=DIRECTION('ref_axis',(0.809016994374948,0.587785252292473,0.));
#7523=DIRECTION('center_axis',(0.,0.,1.));
#7524=DIRECTION('ref_axis',(0.809016994374948,0.587785252292473,0.));
#7525=DIRECTION('',(0.,0.,1.));
#7526=DIRECTION('',(0.,0.,1.));
#7527=DIRECTION('center_axis',(-1.,0.,0.));
#7528=DIRECTION('ref_axis',(0.,-1.,0.));
#7529=DIRECTION('',(0.,-1.,0.));
#7530=DIRECTION('',(0.,0.,1.));
#7531=DIRECTION('center_axis',(0.,0.,1.));
#7532=DIRECTION('ref_axis',(0.809016994374948,0.587785252292473,0.));
#7533=DIRECTION('center_axis',(0.,0.,1.));
#7534=DIRECTION('ref_axis',(0.809016994374948,0.587785252292473,0.));
#7535=DIRECTION('',(0.,0.,1.));
#7536=DIRECTION('center_axis',(0.587785252292473,-0.809016994374947,0.));
#7537=DIRECTION('ref_axis',(0.809016994374947,0.587785252292473,0.));
#7538=DIRECTION('',(0.809016994374947,0.587785252292473,0.));
#7539=DIRECTION('center_axis',(0.,0.,1.));
#7540=DIRECTION('ref_axis',(1.,0.,0.));
#7541=DIRECTION('center_axis',(0.,0.,1.));
#7542=DIRECTION('ref_axis',(1.,0.,0.));
#7543=DIRECTION('center_axis',(0.,0.,1.));
#7544=DIRECTION('ref_axis',(1.,0.,0.));
#7545=DIRECTION('',(0.,0.,-1.));
#7546=DIRECTION('center_axis',(0.,0.,-1.));
#7547=DIRECTION('ref_axis',(1.,0.,0.));
#7548=DIRECTION('center_axis',(0.,0.,1.));
#7549=DIRECTION('ref_axis',(1.,0.,0.));
#7550=DIRECTION('center_axis',(0.,0.,-1.));
#7551=DIRECTION('ref_axis',(1.,0.,0.));
#7552=DIRECTION('center_axis',(0.,0.,1.));
#7553=DIRECTION('ref_axis',(1.,0.,0.));
#7554=DIRECTION('',(0.,0.,-1.));
#7555=DIRECTION('center_axis',(0.,0.,1.));
#7556=DIRECTION('ref_axis',(1.,0.,0.));
#7557=DIRECTION('center_axis',(0.,0.,1.));
#7558=DIRECTION('ref_axis',(1.,0.,0.));
#7559=DIRECTION('',(0.,0.,-1.));
#7560=DIRECTION('center_axis',(0.,0.,1.));
#7561=DIRECTION('ref_axis',(1.,0.,0.));
#8985=CARTESIAN_POINT('',(0.,0.,0.));
#8986=CARTESIAN_POINT('Origin',(1.3,-0.3,3.));
#8987=CARTESIAN_POINT('',(0.953939201416946,-0.3,3.));
#8988=CARTESIAN_POINT('',(0.953939201416946,-0.3,1.8));
#8989=CARTESIAN_POINT('',(0.953939201416946,-0.3,1.8));
#8990=CARTESIAN_POINT('',(1.3,-0.3,3.));
#8991=CARTESIAN_POINT('',(0.7,-0.3,3.));
#8992=CARTESIAN_POINT('',(1.3,-0.3,1.8));
#8993=CARTESIAN_POINT('',(1.3,-0.3,3.));
#8994=CARTESIAN_POINT('',(0.65,-0.3,1.8));
#8995=CARTESIAN_POINT('Origin',(1.3,0.3,3.));
#8996=CARTESIAN_POINT('',(1.3,0.3,3.));
#8997=CARTESIAN_POINT('',(1.3,-0.3,3.));
#8998=CARTESIAN_POINT('',(1.3,0.3,1.8));
#8999=CARTESIAN_POINT('',(1.3,0.3,3.));
#9000=CARTESIAN_POINT('',(1.3,0.15,1.8));
#9001=CARTESIAN_POINT('Origin',(0.7,0.3,3.));
#9002=CARTESIAN_POINT('',(0.953939201416946,0.3,1.8));
#9003=CARTESIAN_POINT('',(0.953939201416946,0.3,3.));
#9004=CARTESIAN_POINT('',(0.953939201416946,0.3,1.8));
#9005=CARTESIAN_POINT('',(0.35,0.3,1.8));
#9006=CARTESIAN_POINT('',(1.3,0.3,3.));
#9007=CARTESIAN_POINT('Origin',(1.,0.,3.));
#9008=CARTESIAN_POINT('Origin',(0.,0.,3.));
#9009=CARTESIAN_POINT('Origin',(0.,0.,1.8));
#9010=CARTESIAN_POINT('',(-5.,-6.12323399573677E-16,1.8));
#9011=CARTESIAN_POINT('Origin',(0.,0.,1.8));
#9012=CARTESIAN_POINT('',(1.01339745962155,-1.95525588832577,1.8));
#9013=CARTESIAN_POINT('',(1.15120561581022,-4.58479215324559,1.8));
#9014=CARTESIAN_POINT('Origin',(-1.49807621135332,-3.40525588832576,1.8));
#9015=CARTESIAN_POINT('',(1.425269253103,-4.70681314616833,1.8));
#9016=CARTESIAN_POINT('',(-0.180963657223493,-3.99167217920436,1.8));
#9017=CARTESIAN_POINT('',(1.27320508075689,-1.80525588832577,1.8));
#9018=CARTESIAN_POINT('Origin',(-1.49807621135332,-3.40525588832576,1.8));
#9019=CARTESIAN_POINT('',(1.18660254037844,-1.85525588832577,1.8));
#9020=CARTESIAN_POINT('',(-1.18660254037845,-1.85525588832576,1.8));
#9021=CARTESIAN_POINT('',(-3.39494366787712,-3.28936938489376,1.8));
#9022=CARTESIAN_POINT('Origin',(-3.69807621135331,-0.405255888325764,1.8));
#9023=CARTESIAN_POINT('',(-3.36358512889683,-3.58772595350424,1.8));
#9024=CARTESIAN_POINT('',(-3.54737133938231,-1.8391169652849,1.8));
#9025=CARTESIAN_POINT('',(-0.926794919243113,-2.00525588832576,1.8));
#9026=CARTESIAN_POINT('Origin',(-3.69807621135332,-0.405255888325764,1.8));
#9027=CARTESIAN_POINT('',(-1.01339745962156,-1.95525588832576,1.8));
#9028=CARTESIAN_POINT('',(-2.2,0.1,1.8));
#9029=CARTESIAN_POINT('',(-4.54614928368735,1.29542276835183,1.8));
#9030=CARTESIAN_POINT('Origin',(-2.2,3.,1.8));
#9031=CARTESIAN_POINT('',(-4.78885438199983,1.11908719266409,1.8));
#9032=CARTESIAN_POINT('',(-3.36640768215882,2.15255521391946,1.8));
#9033=CARTESIAN_POINT('',(-2.2,-0.2,1.8));
#9034=CARTESIAN_POINT('Origin',(-2.2,3.,1.8));
#9035=CARTESIAN_POINT('',(-2.2,-0.0999999999999997,1.8));
#9036=CARTESIAN_POINT('',(-1.01339745962156,1.95525588832577,1.8));
#9037=CARTESIAN_POINT('',(-1.15120561581023,4.58479215324559,1.8));
#9038=CARTESIAN_POINT('Origin',(1.49807621135331,3.40525588832576,1.8));
#9039=CARTESIAN_POINT('',(-1.42526925310301,4.70681314616833,1.8));
#9040=CARTESIAN_POINT('',(0.18096365722349,3.99167217920436,1.8));
#9041=CARTESIAN_POINT('',(-1.27320508075689,1.80525588832577,1.8));
#9042=CARTESIAN_POINT('Origin',(1.49807621135332,3.40525588832576,1.8));
#9043=CARTESIAN_POINT('',(-1.18660254037844,1.85525588832577,1.8));
#9044=CARTESIAN_POINT('',(1.18660254037844,1.85525588832577,1.8));
#9045=CARTESIAN_POINT('',(3.39494366787712,3.28936938489376,1.8));
#9046=CARTESIAN_POINT('Origin',(3.69807621135331,0.405255888325766,1.8));
#9047=CARTESIAN_POINT('',(3.36358512889683,3.58772595350424,1.8));
#9048=CARTESIAN_POINT('',(3.54737133938231,1.8391169652849,1.8));
#9049=CARTESIAN_POINT('',(0.926794919243113,2.00525588832576,1.8));
#9050=CARTESIAN_POINT('Origin',(3.69807621135332,0.405255888325765,1.8));
#9051=CARTESIAN_POINT('',(1.01339745962156,1.95525588832577,1.8));
#9052=CARTESIAN_POINT('',(2.2,-0.1,1.8));
#9053=CARTESIAN_POINT('',(4.54614928368735,-1.29542276835183,1.8));
#9054=CARTESIAN_POINT('Origin',(2.2,-3.,1.8));
#9055=CARTESIAN_POINT('',(4.78885438199983,-1.11908719266409,1.8));
#9056=CARTESIAN_POINT('',(3.36640768215882,-2.15255521391946,1.8));
#9057=CARTESIAN_POINT('',(2.2,0.2,1.8));
#9058=CARTESIAN_POINT('Origin',(2.2,-3.,1.8));
#9059=CARTESIAN_POINT('',(2.2,0.1,1.8));
#9060=CARTESIAN_POINT('',(-1.,-1.22464679914735E-16,1.8));
#9061=CARTESIAN_POINT('Origin',(0.,0.,1.8));
#9062=CARTESIAN_POINT('Origin',(0.,0.,1.8));
#9063=CARTESIAN_POINT('Origin',(-1.49807621135332,-3.40525588832576,0.8));
#9064=CARTESIAN_POINT('',(1.15120561581022,-4.58479215324559,0.8));
#9065=CARTESIAN_POINT('',(1.01339745962155,-1.95525588832577,0.8));
#9066=CARTESIAN_POINT('Origin',(-1.49807621135332,-3.40525588832576,0.8));
#9067=CARTESIAN_POINT('',(1.15120561581022,-4.58479215324559,0.8));
#9068=CARTESIAN_POINT('',(1.01339745962155,-1.95525588832577,0.8));
#9069=CARTESIAN_POINT('Origin',(1.27320508075689,-1.80525588832577,0.8));
#9070=CARTESIAN_POINT('',(1.27320508075689,-1.80525588832577,0.8));
#9071=CARTESIAN_POINT('',(1.27320508075689,-1.80525588832577,0.8));
#9072=CARTESIAN_POINT('',(1.27320508075689,-1.80525588832577,0.8));
#9073=CARTESIAN_POINT('Origin',(-1.49807621135332,-3.40525588832576,0.8));
#9074=CARTESIAN_POINT('',(1.425269253103,-4.70681314616833,0.8));
#9075=CARTESIAN_POINT('Origin',(-1.49807621135332,-3.40525588832576,0.8));
#9076=CARTESIAN_POINT('',(1.425269253103,-4.70681314616833,0.8));
#9077=CARTESIAN_POINT('Origin',(1.15120561581022,-4.58479215324559,0.8));
#9078=CARTESIAN_POINT('',(1.15120561581022,-4.58479215324559,0.8));
#9079=CARTESIAN_POINT('Origin',(1.27288162286168,-3.30011841116898,0.8));
#9080=CARTESIAN_POINT('Origin',(-3.69807621135331,-0.405255888325764,0.8));
#9081=CARTESIAN_POINT('',(-3.39494366787712,-3.28936938489376,0.8));
#9082=CARTESIAN_POINT('',(-1.18660254037845,-1.85525588832576,0.8));
#9083=CARTESIAN_POINT('Origin',(-3.69807621135331,-0.405255888325764,0.8));
#9084=CARTESIAN_POINT('',(-3.39494366787712,-3.28936938489376,0.8));
#9085=CARTESIAN_POINT('',(-1.18660254037845,-1.85525588832576,0.8));
#9086=CARTESIAN_POINT('Origin',(-0.926794919243113,-2.00525588832576,0.8));
#9087=CARTESIAN_POINT('',(-0.926794919243113,-2.00525588832576,0.8));
#9088=CARTESIAN_POINT('',(-0.926794919243113,-2.00525588832576,0.8));
#9089=CARTESIAN_POINT('',(-0.926794919243113,-2.00525588832576,0.8));
#9090=CARTESIAN_POINT('Origin',(-3.69807621135332,-0.405255888325764,0.8));
#9091=CARTESIAN_POINT('',(-3.36358512889683,-3.58772595350424,0.8));
#9092=CARTESIAN_POINT('Origin',(-3.69807621135332,-0.405255888325764,0.8));
#9093=CARTESIAN_POINT('',(-3.36358512889683,-3.58772595350424,0.8));
#9094=CARTESIAN_POINT('Origin',(-3.39494366787712,-3.28936938489376,0.8));
#9095=CARTESIAN_POINT('',(-3.39494366787712,-3.28936938489376,0.8));
#9096=CARTESIAN_POINT('Origin',(-2.22154556813824,-2.75240702699307,0.8));
#9097=CARTESIAN_POINT('Origin',(-2.2,3.,0.8));
#9098=CARTESIAN_POINT('',(-4.54614928368735,1.29542276835183,0.8));
#9099=CARTESIAN_POINT('',(-2.2,0.1,0.8));
#9100=CARTESIAN_POINT('Origin',(-2.2,3.,0.8));
#9101=CARTESIAN_POINT('',(-4.54614928368735,1.29542276835183,0.8));
#9102=CARTESIAN_POINT('',(-2.2,0.1,0.8));
#9103=CARTESIAN_POINT('Origin',(-2.2,-0.2,0.8));
#9104=CARTESIAN_POINT('',(-2.2,-0.2,0.8));
#9105=CARTESIAN_POINT('',(-2.2,-0.2,0.8));
#9106=CARTESIAN_POINT('',(-2.2,-0.2,0.8));
#9107=CARTESIAN_POINT('Origin',(-2.2,3.,0.8));
#9108=CARTESIAN_POINT('',(-4.78885438199983,1.11908719266409,0.8));
#9109=CARTESIAN_POINT('Origin',(-2.2,3.,0.8));
#9110=CARTESIAN_POINT('',(-4.78885438199983,1.11908719266409,0.8));
#9111=CARTESIAN_POINT('Origin',(-4.54614928368735,1.29542276835183,0.8));
#9112=CARTESIAN_POINT('',(-4.54614928368735,1.29542276835183,0.8));
#9113=CARTESIAN_POINT('Origin',(-3.49442719099992,0.547711384175914,0.8));
#9114=CARTESIAN_POINT('Origin',(1.49807621135331,3.40525588832576,0.8));
#9115=CARTESIAN_POINT('',(-1.15120561581023,4.58479215324559,0.8));
#9116=CARTESIAN_POINT('',(-1.01339745962156,1.95525588832577,0.8));
#9117=CARTESIAN_POINT('Origin',(1.49807621135331,3.40525588832576,0.8));
#9118=CARTESIAN_POINT('',(-1.15120561581023,4.58479215324559,0.8));
#9119=CARTESIAN_POINT('',(-1.01339745962156,1.95525588832577,0.8));
#9120=CARTESIAN_POINT('Origin',(-1.27320508075689,1.80525588832577,0.8));
#9121=CARTESIAN_POINT('',(-1.27320508075689,1.80525588832577,0.8));
#9122=CARTESIAN_POINT('',(-1.27320508075689,1.80525588832577,0.8));
#9123=CARTESIAN_POINT('',(-1.27320508075689,1.80525588832577,0.8));
#9124=CARTESIAN_POINT('Origin',(1.49807621135332,3.40525588832576,0.8));
#9125=CARTESIAN_POINT('',(-1.42526925310301,4.70681314616833,0.8));
#9126=CARTESIAN_POINT('Origin',(1.49807621135332,3.40525588832576,0.8));
#9127=CARTESIAN_POINT('',(-1.42526925310301,4.70681314616833,0.8));
#9128=CARTESIAN_POINT('Origin',(-1.15120561581023,4.58479215324559,0.8));
#9129=CARTESIAN_POINT('',(-1.15120561581023,4.58479215324559,0.8));
#9130=CARTESIAN_POINT('Origin',(-1.27288162286168,3.30011841116898,0.8));
#9131=CARTESIAN_POINT('Origin',(3.69807621135331,0.405255888325766,0.8));
#9132=CARTESIAN_POINT('',(3.39494366787712,3.28936938489376,0.8));
#9133=CARTESIAN_POINT('',(1.18660254037844,1.85525588832577,0.8));
#9134=CARTESIAN_POINT('Origin',(3.69807621135331,0.405255888325766,0.8));
#9135=CARTESIAN_POINT('',(3.39494366787712,3.28936938489376,0.8));
#9136=CARTESIAN_POINT('',(1.18660254037844,1.85525588832577,0.8));
#9137=CARTESIAN_POINT('Origin',(0.926794919243113,2.00525588832576,0.8));
#9138=CARTESIAN_POINT('',(0.926794919243113,2.00525588832576,0.8));
#9139=CARTESIAN_POINT('',(0.926794919243113,2.00525588832576,0.8));
#9140=CARTESIAN_POINT('',(0.926794919243113,2.00525588832576,0.8));
#9141=CARTESIAN_POINT('Origin',(3.69807621135332,0.405255888325765,0.8));
#9142=CARTESIAN_POINT('',(3.36358512889683,3.58772595350424,0.8));
#9143=CARTESIAN_POINT('Origin',(3.69807621135332,0.405255888325765,0.8));
#9144=CARTESIAN_POINT('',(3.36358512889683,3.58772595350424,0.8));
#9145=CARTESIAN_POINT('Origin',(3.39494366787712,3.28936938489376,0.8));
#9146=CARTESIAN_POINT('',(3.39494366787712,3.28936938489376,0.8));
#9147=CARTESIAN_POINT('Origin',(2.22154556813824,2.75240702699307,0.8));
#9148=CARTESIAN_POINT('Origin',(2.2,-3.,0.8));
#9149=CARTESIAN_POINT('',(4.54614928368735,-1.29542276835183,0.8));
#9150=CARTESIAN_POINT('',(2.2,-0.1,0.8));
#9151=CARTESIAN_POINT('Origin',(2.2,-3.,0.8));
#9152=CARTESIAN_POINT('',(4.54614928368735,-1.29542276835183,0.8));
#9153=CARTESIAN_POINT('',(2.2,-0.1,0.8));
#9154=CARTESIAN_POINT('Origin',(2.2,0.2,0.8));
#9155=CARTESIAN_POINT('',(2.2,0.2,0.8));
#9156=CARTESIAN_POINT('',(2.2,0.2,0.8));
#9157=CARTESIAN_POINT('',(2.2,0.2,0.8));
#9158=CARTESIAN_POINT('Origin',(2.2,-3.,0.8));
#9159=CARTESIAN_POINT('',(4.78885438199983,-1.11908719266409,0.8));
#9160=CARTESIAN_POINT('Origin',(2.2,-3.,0.8));
#9161=CARTESIAN_POINT('',(4.78885438199983,-1.11908719266409,0.8));
#9162=CARTESIAN_POINT('Origin',(4.54614928368735,-1.29542276835183,0.8));
#9163=CARTESIAN_POINT('',(4.54614928368735,-1.29542276835183,0.8));
#9164=CARTESIAN_POINT('Origin',(3.49442719099992,-0.547711384175914,0.8));
#9165=CARTESIAN_POINT('Origin',(0.,0.,2.2));
#9166=CARTESIAN_POINT('',(-1.5,-1.83697019872103E-16,3.2));
#9167=CARTESIAN_POINT('Origin',(0.,0.,3.2));
#9168=CARTESIAN_POINT('',(-1.5,-1.83697019872103E-16,2.2));
#9169=CARTESIAN_POINT('',(-1.5,-1.83697019872103E-16,2.2));
#9170=CARTESIAN_POINT('Origin',(0.,0.,2.2));
#9171=CARTESIAN_POINT('Origin',(0.,0.,3.2));
#9172=CARTESIAN_POINT('',(-1.,-1.22464679914735E-16,3.2));
#9173=CARTESIAN_POINT('Origin',(0.,0.,3.2));
#9174=CARTESIAN_POINT('Origin',(0.,0.,1.8));
#9175=CARTESIAN_POINT('',(-1.,-1.22464679914735E-16,1.8));
#9176=CARTESIAN_POINT('Origin',(0.,0.,1.8));
#9177=CARTESIAN_POINT('',(-5.,-6.12323399573677E-16,2.2));
#9178=CARTESIAN_POINT('Origin',(0.,0.,2.2));
#9179=CARTESIAN_POINT('',(-5.,-6.12323399573677E-16,1.8));
#9180=CARTESIAN_POINT('Origin',(0.,0.,2.2));
#16649=UNCERTAINTY_MEASURE_WITH_UNIT(LENGTH_MEASURE(0.001),#16688,
'DISTANCE_ACCURACY_VALUE',
'Maximum model space distance between geometric entities at asserted c
onnectivities');
#16666=UNCERTAINTY_MEASURE_WITH_UNIT(LENGTH_MEASURE(0.001),#16688,
'DISTANCE_ACCURACY_VALUE',
'Maximum model space distance between geometric entities at asserted c
onnectivities');
#16670=(
GEOMETRIC_REPRESENTATION_CONTEXT(3)
GLOBAL_UNCERTAINTY_ASSIGNED_CONTEXT((#16649))
GLOBAL_UNIT_ASSIGNED_CONTEXT((#16688,#16690,#16691))
REPRESENTATION_CONTEXT('','3D')
);
#16687=(
GEOMETRIC_REPRESENTATION_CONTEXT(3)
GLOBAL_UNCERTAINTY_ASSIGNED_CONTEXT((#16666))
GLOBAL_UNIT_ASSIGNED_CONTEXT((#16688,#16690,#16691))
REPRESENTATION_CONTEXT('','3D')
);
#16688=(
LENGTH_UNIT()
NAMED_UNIT(*)
SI_UNIT(.CENTI.,.METRE.)
);
#16690=(
NAMED_UNIT(*)
PLANE_ANGLE_UNIT()
SI_UNIT($,.RADIAN.)
);
#16691=(
NAMED_UNIT(*)
SI_UNIT($,.STERADIAN.)
SOLID_ANGLE_UNIT()
);
#16695=SHAPE_DEFINITION_REPRESENTATION(#16715,#16766);
#16715=PRODUCT_DEFINITION_SHAPE('',$,#16787);
#16766=SHAPE_REPRESENTATION('',(#6480),#16670);
#16783=PRODUCT_DEFINITION_CONTEXT('part definition',#16845,'design');
#16787=PRODUCT_DEFINITION('Radial impeller','Radial impeller',#16807,#16783);
#16807=PRODUCT_DEFINITION_FORMATION('',$,#16850);
#16845=APPLICATION_CONTEXT(
'Core Data for Automotive Mechanical Design Process');
#16846=PRODUCT_CONTEXT('part definition',#16845,'mechanical');
#16850=PRODUCT('Radial impeller','Radial impeller',$,(#16846));
#16870=PRESENTATION_STYLE_ASSIGNMENT((#16885));
#16885=SURFACE_STYLE_USAGE(.BOTH.,#16900);
#16900=SURFACE_SIDE_STYLE('',(#16915));
#16915=SURFACE_STYLE_FILL_AREA(#16930);
#16930=FILL_AREA_STYLE('Light blue',(#16945));
#16945=FILL_AREA_STYLE_COLOUR('Light blue',#16960);
#16960=COLOUR_RGB('Light blue',0.662745098039216,0.831372549019608,0.949019607843137);
ENDSEC;
END-ISO-10303-21;
